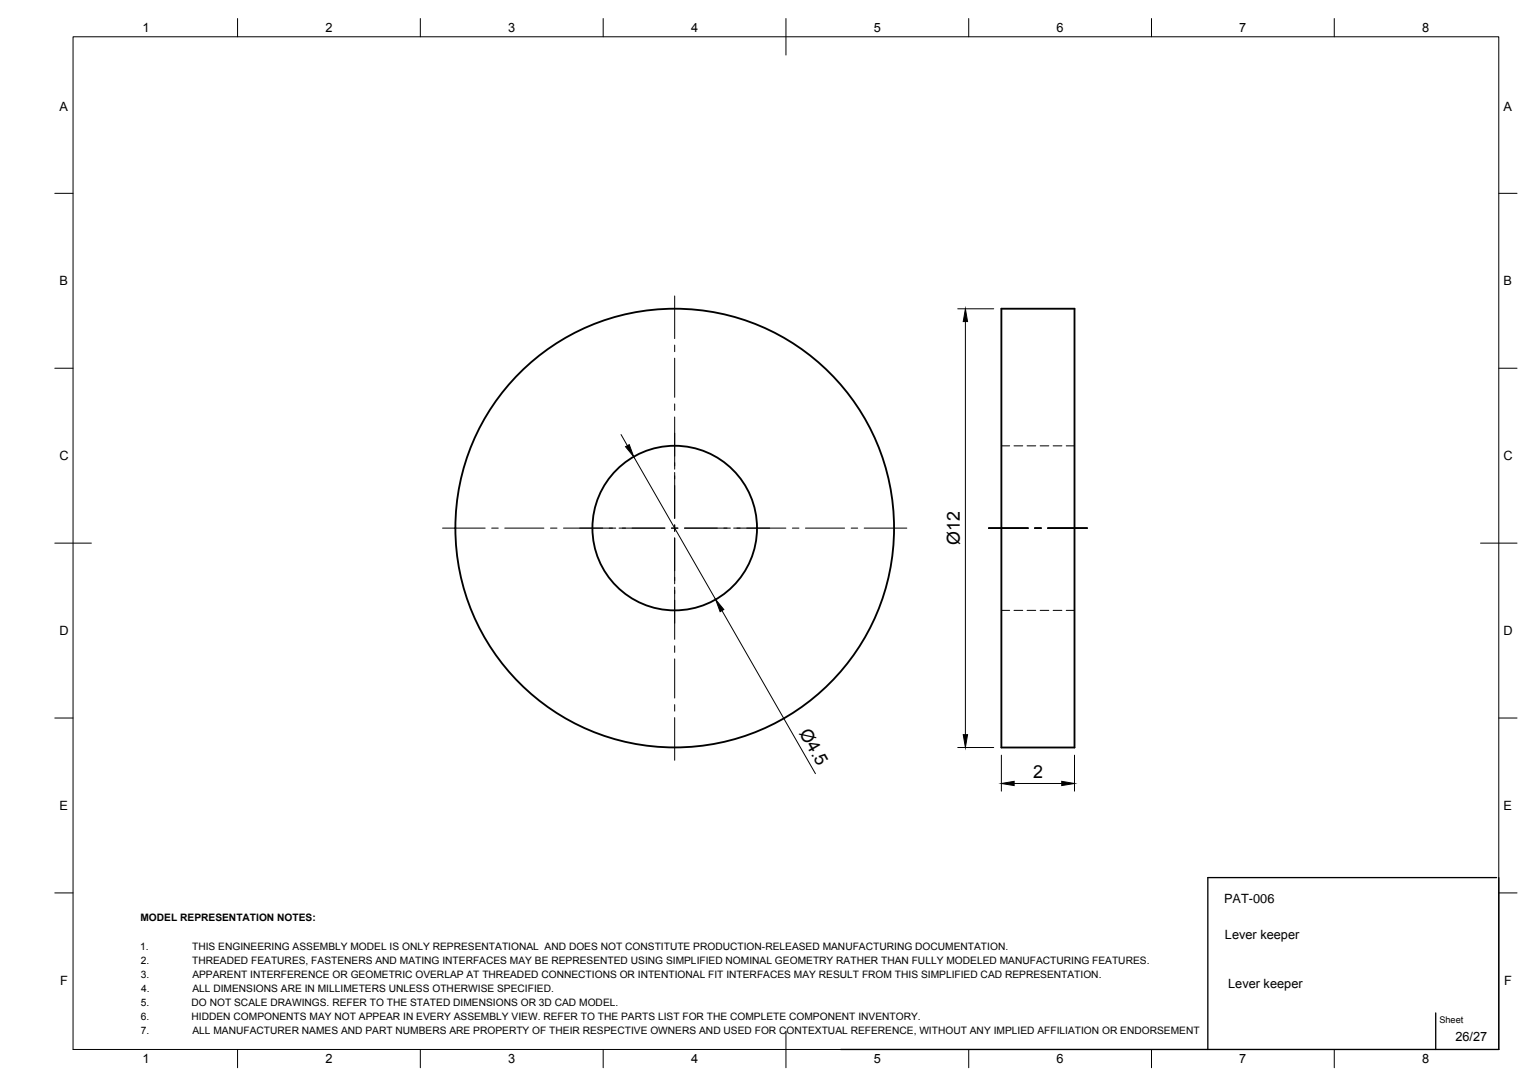
ISO-10303-21;
HEADER;
/* Generated by software containing ST-Developer
 * from STEP Tools, Inc. (www.steptools.com) 
 */

FILE_DESCRIPTION(
/* description */ ('Ball-type isolation valve (generic)'),
/* implementation_level */ '2;1');

FILE_NAME(
/* name */ 'Lever keeper.step',
/* time_stamp */ '2026-10-27T10:53:05-07:00',
/* author */ (''),
/* organization */ (''),
/* preprocessor_version */ 'ST-DEVELOPER v20.2',
/* originating_system */ 'Autodesk Translation Framework v15.17.0.0',
/* authorisation */ '');

FILE_SCHEMA (('AUTOMOTIVE_DESIGN { 1 0 10303 214 3 1 1 }'));
ENDSEC;

DATA;
#10=MECHANICAL_DESIGN_GEOMETRIC_PRESENTATION_REPRESENTATION('',(#300),#7425);
#248=SHAPE_REPRESENTATION_RELATIONSHIP('SRR','None',#7559,#274);
#274=ADVANCED_BREP_SHAPE_REPRESENTATION('',(#324),#7422);
#300=STYLED_ITEM('',(#7737),#324);
#324=MANIFOLD_SOLID_BREP('Body1',#4107);
#416=FACE_BOUND('',#1139,.T.);
#417=FACE_BOUND('',#1141,.T.);
#560=PLANE('',#4855);
#561=PLANE('',#4856);
#802=FACE_OUTER_BOUND('',#1136,.T.);
#803=FACE_OUTER_BOUND('',#1137,.T.);
#804=FACE_OUTER_BOUND('',#1138,.T.);
#805=FACE_OUTER_BOUND('',#1140,.T.);
#1136=EDGE_LOOP('',(#3669,#3670,#3671,#3672));
#1137=EDGE_LOOP('',(#3673,#3674,#3675,#3676));
#1138=EDGE_LOOP('',(#3677));
#1139=EDGE_LOOP('',(#3678));
#1140=EDGE_LOOP('',(#3679));
#1141=EDGE_LOOP('',(#3680));
#1436=LINE('',#7255,#1744);
#1437=LINE('',#7261,#1745);
#1744=VECTOR('',#6073,0.225);
#1745=VECTOR('',#6080,0.6);
#1945=CIRCLE('',#4850,0.225);
#1946=CIRCLE('',#4851,0.225);
#1947=CIRCLE('',#4853,0.6);
#1948=CIRCLE('',#4854,0.6);
#2249=VERTEX_POINT('',#7252);
#2250=VERTEX_POINT('',#7254);
#2251=VERTEX_POINT('',#7258);
#2252=VERTEX_POINT('',#7260);
#2727=EDGE_CURVE('',#2249,#2249,#1945,.T.);
#2728=EDGE_CURVE('',#2249,#2250,#1436,.T.);
#2729=EDGE_CURVE('',#2250,#2250,#1946,.T.);
#2730=EDGE_CURVE('',#2251,#2251,#1947,.T.);
#2731=EDGE_CURVE('',#2251,#2252,#1437,.T.);
#2732=EDGE_CURVE('',#2252,#2252,#1948,.T.);
#3669=ORIENTED_EDGE('',*,*,#2727,.F.);
#3670=ORIENTED_EDGE('',*,*,#2728,.T.);
#3671=ORIENTED_EDGE('',*,*,#2729,.T.);
#3672=ORIENTED_EDGE('',*,*,#2728,.F.);
#3673=ORIENTED_EDGE('',*,*,#2730,.F.);
#3674=ORIENTED_EDGE('',*,*,#2731,.T.);
#3675=ORIENTED_EDGE('',*,*,#2732,.T.);
#3676=ORIENTED_EDGE('',*,*,#2731,.F.);
#3677=ORIENTED_EDGE('',*,*,#2730,.T.);
#3678=ORIENTED_EDGE('',*,*,#2727,.T.);
#3679=ORIENTED_EDGE('',*,*,#2732,.F.);
#3680=ORIENTED_EDGE('',*,*,#2729,.F.);
#3829=CYLINDRICAL_SURFACE('',#4849,0.225);
#3830=CYLINDRICAL_SURFACE('',#4852,0.6);
#4056=ADVANCED_FACE('',(#802),#3829,.F.);
#4057=ADVANCED_FACE('',(#803),#3830,.T.);
#4058=ADVANCED_FACE('',(#804,#416),#560,.T.);
#4059=ADVANCED_FACE('',(#805,#417),#561,.F.);
#4107=CLOSED_SHELL('',(#4056,#4057,#4058,#4059));
#4848=AXIS2_PLACEMENT_3D('',#7250,#6067,#6068);
#4849=AXIS2_PLACEMENT_3D('',#7251,#6069,#6070);
#4850=AXIS2_PLACEMENT_3D('',#7253,#6071,#6072);
#4851=AXIS2_PLACEMENT_3D('',#7256,#6074,#6075);
#4852=AXIS2_PLACEMENT_3D('',#7257,#6076,#6077);
#4853=AXIS2_PLACEMENT_3D('',#7259,#6078,#6079);
#4854=AXIS2_PLACEMENT_3D('',#7262,#6081,#6082);
#4855=AXIS2_PLACEMENT_3D('',#7263,#6083,#6084);
#4856=AXIS2_PLACEMENT_3D('',#7264,#6085,#6086);
#6067=DIRECTION('axis',(0.,0.,1.));
#6068=DIRECTION('refdir',(1.,0.,0.));
#6069=DIRECTION('center_axis',(0.,0.,1.));
#6070=DIRECTION('ref_axis',(1.,0.,0.));
#6071=DIRECTION('center_axis',(0.,0.,-1.));
#6072=DIRECTION('ref_axis',(1.,0.,0.));
#6073=DIRECTION('',(0.,0.,-1.));
#6074=DIRECTION('center_axis',(0.,0.,-1.));
#6075=DIRECTION('ref_axis',(1.,0.,0.));
#6076=DIRECTION('center_axis',(0.,0.,1.));
#6077=DIRECTION('ref_axis',(1.,0.,0.));
#6078=DIRECTION('center_axis',(0.,0.,1.));
#6079=DIRECTION('ref_axis',(1.,0.,0.));
#6080=DIRECTION('',(0.,0.,-1.));
#6081=DIRECTION('center_axis',(0.,0.,1.));
#6082=DIRECTION('ref_axis',(1.,0.,0.));
#6083=DIRECTION('center_axis',(0.,0.,1.));
#6084=DIRECTION('ref_axis',(1.,0.,0.));
#6085=DIRECTION('center_axis',(0.,0.,1.));
#6086=DIRECTION('ref_axis',(1.,0.,0.));
#7250=CARTESIAN_POINT('',(0.,0.,0.));
#7251=CARTESIAN_POINT('Origin',(0.,0.,9.4));
#7252=CARTESIAN_POINT('',(-0.225,-2.75545529808154E-17,9.6));
#7253=CARTESIAN_POINT('Origin',(0.,0.,9.6));
#7254=CARTESIAN_POINT('',(-0.225,-2.75545529808154E-17,9.4));
#7255=CARTESIAN_POINT('',(-0.225,-2.75545529808154E-17,9.4));
#7256=CARTESIAN_POINT('Origin',(0.,0.,9.4));
#7257=CARTESIAN_POINT('Origin',(0.,0.,9.4));
#7258=CARTESIAN_POINT('',(-0.6,-7.34788079488412E-17,9.6));
#7259=CARTESIAN_POINT('Origin',(0.,0.,9.6));
#7260=CARTESIAN_POINT('',(-0.6,-7.34788079488412E-17,9.4));
#7261=CARTESIAN_POINT('',(-0.6,-7.34788079488412E-17,9.4));
#7262=CARTESIAN_POINT('Origin',(0.,0.,9.4));
#7263=CARTESIAN_POINT('Origin',(0.,0.,9.6));
#7264=CARTESIAN_POINT('Origin',(0.,0.,9.4));
#7392=UNCERTAINTY_MEASURE_WITH_UNIT(LENGTH_MEASURE(0.001),#7426,
'DISTANCE_ACCURACY_VALUE',
'Maximum model space distance between geometric entities at asserted c
onnectivities');
#7395=UNCERTAINTY_MEASURE_WITH_UNIT(LENGTH_MEASURE(0.001),#7426,
'DISTANCE_ACCURACY_VALUE',
'Maximum model space distance between geometric entities at asserted c
onnectivities');
#7422=(
GEOMETRIC_REPRESENTATION_CONTEXT(3)
GLOBAL_UNCERTAINTY_ASSIGNED_CONTEXT((#7392))
GLOBAL_UNIT_ASSIGNED_CONTEXT((#7426,#7428,#7429))
REPRESENTATION_CONTEXT('','3D')
);
#7425=(
GEOMETRIC_REPRESENTATION_CONTEXT(3)
GLOBAL_UNCERTAINTY_ASSIGNED_CONTEXT((#7395))
GLOBAL_UNIT_ASSIGNED_CONTEXT((#7426,#7428,#7429))
REPRESENTATION_CONTEXT('','3D')
);
#7426=(
LENGTH_UNIT()
NAMED_UNIT(*)
SI_UNIT(.CENTI.,.METRE.)
);
#7428=(
NAMED_UNIT(*)
PLANE_ANGLE_UNIT()
SI_UNIT($,.RADIAN.)
);
#7429=(
NAMED_UNIT(*)
SI_UNIT($,.STERADIAN.)
SOLID_ANGLE_UNIT()
);
#7456=SHAPE_DEFINITION_REPRESENTATION(#7522,#7559);
#7522=PRODUCT_DEFINITION_SHAPE('',$,#7589);
#7559=SHAPE_REPRESENTATION('',(#4848),#7422);
#7562=PRODUCT_DEFINITION_CONTEXT('part definition',#7651,'design');
#7589=PRODUCT_DEFINITION('Lever keeper','Lever keeper',#7618,#7562);
#7618=PRODUCT_DEFINITION_FORMATION('',$,#7679);
#7651=APPLICATION_CONTEXT(
'Core Data for Automotive Mechanical Design Process');
#7652=PRODUCT_CONTEXT('part definition',#7651,'mechanical');
#7679=PRODUCT('Lever keeper','Lever keeper','Lever keeper',(#7652));
#7731=COLOUR_RGB('Sky Blue',0.24,0.69,0.87);
#7732=FILL_AREA_STYLE_COLOUR('',#7731);
#7733=FILL_AREA_STYLE('',(#7732));
#7734=SURFACE_STYLE_FILL_AREA(#7733);
#7735=SURFACE_SIDE_STYLE('',(#7734));
#7736=SURFACE_STYLE_USAGE(.BOTH.,#7735);
#7737=PRESENTATION_STYLE_ASSIGNMENT((#7736));
ENDSEC;
END-ISO-10303-21;
